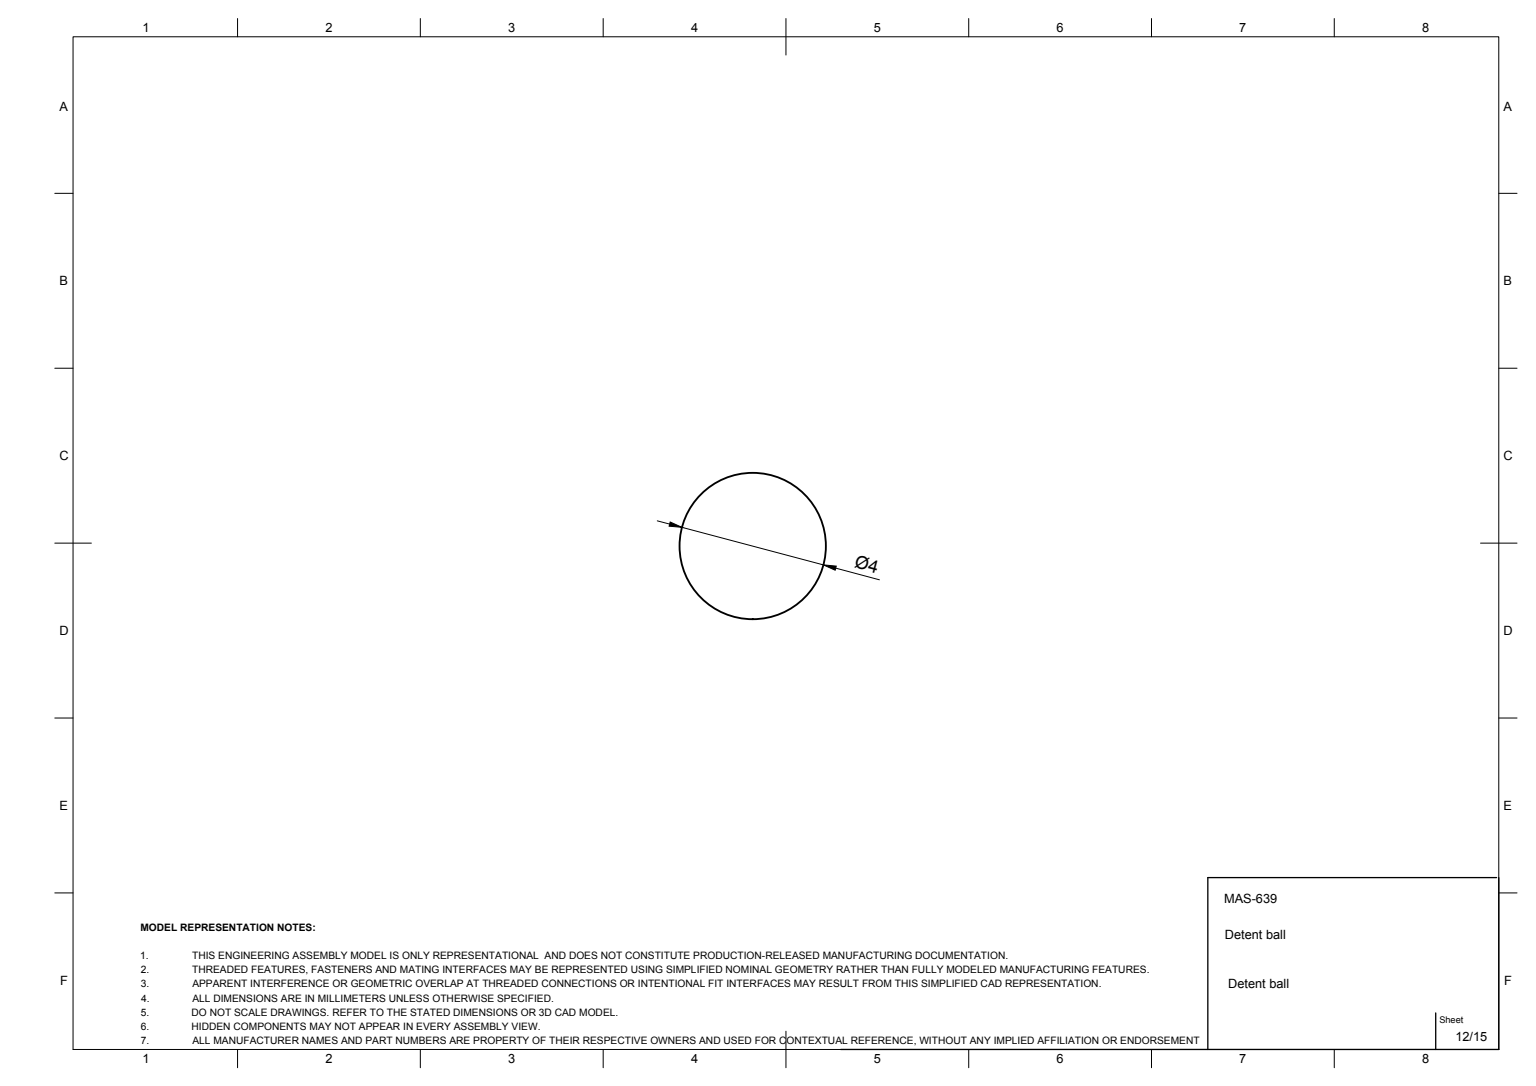
ISO-10303-21;
HEADER;
/* Generated by software containing ST-Developer
 * from STEP Tools, Inc. (www.steptools.com) 
 */

FILE_DESCRIPTION(
/* description */ ('Independent maintained push-to-latch/pull-to-reset mushroom-operator 
CAD. Two opposed spring-loaded ball detents in turned circular seats b
ias both travel stops; direct normally-closed bridge opens6mm when pre
ssed. Rounded palm/pull rim, captured head screw, removable detent clo
sures, native Coil spring families, insulated shared terminals and ord
inary machining features. Manual geometric states and ideal same-mater
ial spring-energy direction only; no electrical/safety certification, 
force/contact dynamics, wear, load or life rating. Requested blue/gray
 visual palette, not safety identification. External wiring/anchors an
d application engineering omitted.'),
/* implementation_level */ '2;1');

FILE_NAME(
/* name */ 'Detent ball.step',
/* time_stamp */ '2026-11-08T17:54:26-08:00',
/* author */ (''),
/* organization */ (''),
/* preprocessor_version */ 'ST-DEVELOPER v20.2',
/* originating_system */ 'Autodesk Translation Framework v15.17.0.0',
/* authorisation */ '');

FILE_SCHEMA (('AUTOMOTIVE_DESIGN { 1 0 10303 214 3 1 1 }'));
ENDSEC;

DATA;
#10=MECHANICAL_DESIGN_GEOMETRIC_PRESENTATION_REPRESENTATION('',(#200),#43980);
#151=SPHERICAL_SURFACE('',#12036,0.2);
#166=SHAPE_REPRESENTATION_RELATIONSHIP('SRR','None',#44066,#183);
#183=ADVANCED_BREP_SHAPE_REPRESENTATION('',(#217),#43973);
#200=STYLED_ITEM('',(#44158),#217);
#217=MANIFOLD_SOLID_BREP('Body1',#11241);
#941=FACE_OUTER_BOUND('',#1627,.T.);
#1627=EDGE_LOOP('',(#9323,#9324));
#1957=CIRCLE('',#12037,0.2);
#4912=VERTEX_POINT('',#35893);
#4913=VERTEX_POINT('',#35894);
#6431=EDGE_CURVE('',#4912,#4913,#1957,.T.);
#9323=ORIENTED_EDGE('',*,*,#6431,.T.);
#9324=ORIENTED_EDGE('',*,*,#6431,.F.);
#11066=ADVANCED_FACE('',(#941),#151,.T.);
#11241=CLOSED_SHELL('',(#11066));
#12035=AXIS2_PLACEMENT_3D('',#35891,#13923,#13924);
#12036=AXIS2_PLACEMENT_3D('',#35892,#13925,#13926);
#12037=AXIS2_PLACEMENT_3D('',#35895,#13927,#13928);
#13923=DIRECTION('axis',(0.,0.,1.));
#13924=DIRECTION('refdir',(1.,0.,0.));
#13925=DIRECTION('center_axis',(6.12323399573677E-17,0.,1.));
#13926=DIRECTION('ref_axis',(1.,0.,0.));
#13927=DIRECTION('center_axis',(1.22464679914735E-16,-1.,0.));
#13928=DIRECTION('ref_axis',(-1.,-1.22464679914735E-16,0.));
#35891=CARTESIAN_POINT('',(0.,0.,0.));
#35892=CARTESIAN_POINT('Origin',(0.,0.,0.));
#35893=CARTESIAN_POINT('',(-1.22464679914735E-17,-1.49975978266186E-33,
0.2));
#35894=CARTESIAN_POINT('',(-1.22464679914735E-17,-1.49975978266186E-33,
-0.2));
#35895=CARTESIAN_POINT('Origin',(0.,0.,0.));
#43954=UNCERTAINTY_MEASURE_WITH_UNIT(LENGTH_MEASURE(0.001),#43981,
'DISTANCE_ACCURACY_VALUE',
'Maximum model space distance between geometric entities at asserted c
onnectivities');
#43961=UNCERTAINTY_MEASURE_WITH_UNIT(LENGTH_MEASURE(0.001),#43981,
'DISTANCE_ACCURACY_VALUE',
'Maximum model space distance between geometric entities at asserted c
onnectivities');
#43973=(
GEOMETRIC_REPRESENTATION_CONTEXT(3)
GLOBAL_UNCERTAINTY_ASSIGNED_CONTEXT((#43954))
GLOBAL_UNIT_ASSIGNED_CONTEXT((#43981,#43983,#43984))
REPRESENTATION_CONTEXT('','3D')
);
#43980=(
GEOMETRIC_REPRESENTATION_CONTEXT(3)
GLOBAL_UNCERTAINTY_ASSIGNED_CONTEXT((#43961))
GLOBAL_UNIT_ASSIGNED_CONTEXT((#43981,#43983,#43984))
REPRESENTATION_CONTEXT('','3D')
);
#43981=(
LENGTH_UNIT()
NAMED_UNIT(*)
SI_UNIT(.CENTI.,.METRE.)
);
#43983=(
NAMED_UNIT(*)
PLANE_ANGLE_UNIT()
SI_UNIT($,.RADIAN.)
);
#43984=(
NAMED_UNIT(*)
SI_UNIT($,.STERADIAN.)
SOLID_ANGLE_UNIT()
);
#43996=SHAPE_DEFINITION_REPRESENTATION(#44014,#44066);
#44014=PRODUCT_DEFINITION_SHAPE('',$,#44085);
#44066=SHAPE_REPRESENTATION('',(#12035),#43973);
#44073=PRODUCT_DEFINITION_CONTEXT('part definition',#44129,'design');
#44085=PRODUCT_DEFINITION('Detent ball','Detent ball',#44103,#44073);
#44103=PRODUCT_DEFINITION_FORMATION('',$,#44142);
#44129=APPLICATION_CONTEXT(
'Core Data for Automotive Mechanical Design Process');
#44130=PRODUCT_CONTEXT('part definition',#44129,'mechanical');
#44142=PRODUCT('Detent ball','Detent ball','Detent ball',(#44130));
#44158=PRESENTATION_STYLE_ASSIGNMENT((#44170));
#44170=SURFACE_STYLE_USAGE(.BOTH.,#44182);
#44182=SURFACE_SIDE_STYLE('',(#44194));
#44194=SURFACE_STYLE_FILL_AREA(#44206);
#44206=FILL_AREA_STYLE('Ball gray',(#44218));
#44218=FILL_AREA_STYLE_COLOUR('Ball gray',#44230);
#44230=COLOUR_RGB('Ball gray',0.725490196078431,0.752941176470588,0.792156862745098);
ENDSEC;
END-ISO-10303-21;
